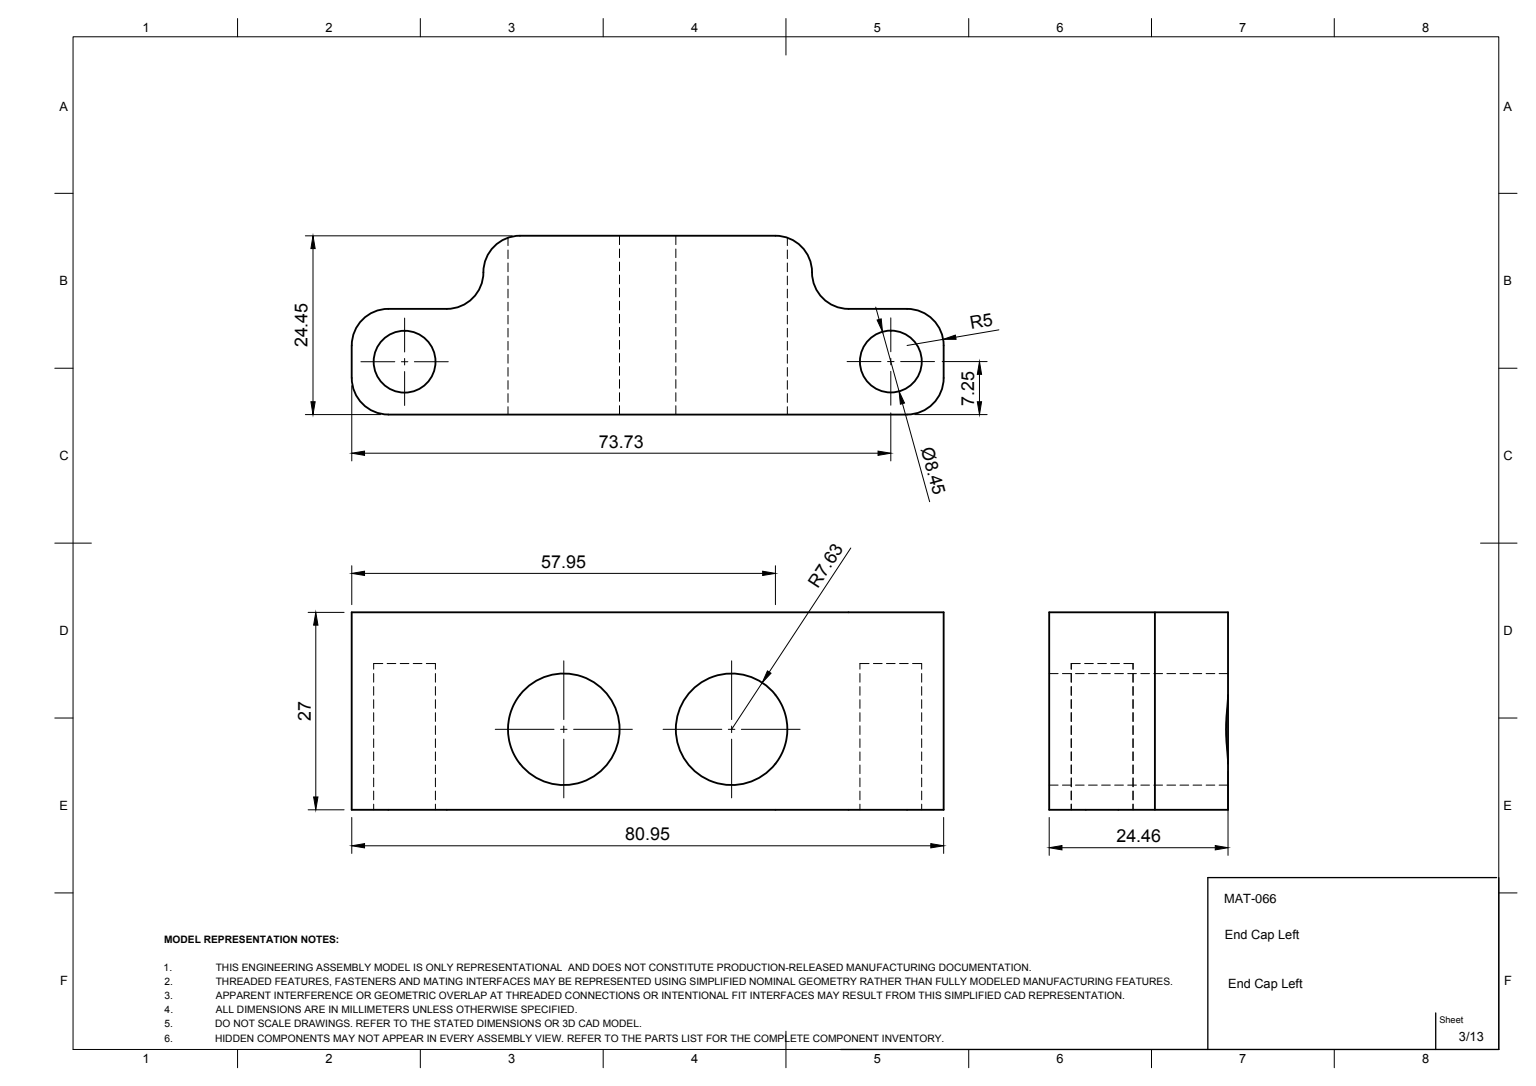
ISO-10303-21;
HEADER;
/* Generated by software containing ST-Developer
 * from STEP Tools, Inc. (www.steptools.com) 
 */

FILE_DESCRIPTION(
/* description */ ('CAx-IF Rec.Pracs.---Representation and Presentation of Product Manufa
cturing Information (PMI)---4.0---2014-10-13'),
/* implementation_level */ '2;1');

FILE_NAME(
/* name */ 'End Cap Left.step',
/* time_stamp */ '2026-10-24T15:58:00-07:00',
/* author */ (''),
/* organization */ (''),
/* preprocessor_version */ 'ST-DEVELOPER v20.2',
/* originating_system */ 'Autodesk Translation Framework v15.17.0.0',
/* authorisation */ '');

FILE_SCHEMA (('AP242_MANAGED_MODEL_BASED_3D_ENGINEERING_MIM_LF { 1 0 10303 442 2 1 4 }'));
ENDSEC;

DATA;
#10=MECHANICAL_DESIGN_GEOMETRIC_PRESENTATION_REPRESENTATION('',(#129),#8944);
#111=SHAPE_REPRESENTATION_RELATIONSHIP('SRR','None',#8993,#120);
#120=ADVANCED_BREP_SHAPE_REPRESENTATION('',(#138),#8934);
#129=STYLED_ITEM('',(#9052),#138);
#138=MANIFOLD_SOLID_BREP('Body1',#5150);
#147=B_SPLINE_CURVE_WITH_KNOTS('',3,(#7501,#7502,#7503,#7504,#7505,#7506),
 .UNSPECIFIED.,.F.,.F.,(4,2,4),(3.46797062946804,3.66737221611079,3.95578831781598),
 .UNSPECIFIED.);
#148=B_SPLINE_CURVE_WITH_KNOTS('',3,(#7507,#7508,#7509,#7510,#7511,#7512),
 .UNSPECIFIED.,.F.,.F.,(4,2,4),(3.95578831781598,4.24420441952117,4.44360600616391),
 .UNSPECIFIED.);
#149=B_SPLINE_CURVE_WITH_KNOTS('',3,(#7515,#7516,#7517,#7518,#7519,#7520,
#7521,#7522,#7523,#7524),.UNSPECIFIED.,.F.,.F.,(4,2,2,2,4),(-4.44360600616391,
-4.24420441952117,-3.95578831781597,-3.66737221611078,-3.46797062946804),
 .UNSPECIFIED.);
#153=CYLINDRICAL_SURFACE('',#5276,0.004225);
#154=CYLINDRICAL_SURFACE('',#5280,0.004225);
#155=CYLINDRICAL_SURFACE('',#5294,0.005);
#156=CYLINDRICAL_SURFACE('',#5295,0.005);
#157=CYLINDRICAL_SURFACE('',#5296,0.005);
#158=CYLINDRICAL_SURFACE('',#5297,0.005);
#159=CYLINDRICAL_SURFACE('',#5302,0.007625);
#160=CYLINDRICAL_SURFACE('',#5303,0.007625);
#161=CYLINDRICAL_SURFACE('',#5304,0.005);
#162=CYLINDRICAL_SURFACE('',#5305,0.005);
#163=CYLINDRICAL_SURFACE('',#5306,0.005);
#164=CYLINDRICAL_SURFACE('',#5307,0.005);
#238=FACE_BOUND('',#581,.T.);
#239=FACE_BOUND('',#582,.T.);
#240=FACE_BOUND('',#588,.T.);
#241=FACE_BOUND('',#589,.T.);
#308=FACE_OUTER_BOUND('',#577,.T.);
#309=FACE_OUTER_BOUND('',#578,.T.);
#310=FACE_OUTER_BOUND('',#579,.T.);
#311=FACE_OUTER_BOUND('',#580,.T.);
#312=FACE_OUTER_BOUND('',#583,.T.);
#313=FACE_OUTER_BOUND('',#584,.T.);
#314=FACE_OUTER_BOUND('',#585,.T.);
#315=FACE_OUTER_BOUND('',#586,.T.);
#316=FACE_OUTER_BOUND('',#587,.T.);
#317=FACE_OUTER_BOUND('',#590,.T.);
#318=FACE_OUTER_BOUND('',#591,.T.);
#319=FACE_OUTER_BOUND('',#592,.T.);
#320=FACE_OUTER_BOUND('',#593,.T.);
#321=FACE_OUTER_BOUND('',#594,.T.);
#322=FACE_OUTER_BOUND('',#595,.T.);
#323=FACE_OUTER_BOUND('',#596,.T.);
#324=FACE_OUTER_BOUND('',#597,.T.);
#325=FACE_OUTER_BOUND('',#598,.T.);
#326=FACE_OUTER_BOUND('',#599,.T.);
#327=FACE_OUTER_BOUND('',#600,.T.);
#328=FACE_OUTER_BOUND('',#601,.T.);
#329=FACE_OUTER_BOUND('',#602,.T.);
#577=EDGE_LOOP('',(#3275,#3276,#3277,#3278,#3279,#3280,#3281,#3282,#3283,
#3284,#3285,#3286,#3287,#3288));
#578=EDGE_LOOP('',(#3289,#3290,#3291,#3292));
#579=EDGE_LOOP('',(#3293,#3294,#3295,#3296));
#580=EDGE_LOOP('',(#3297,#3298,#3299,#3300));
#581=EDGE_LOOP('',(#3301));
#582=EDGE_LOOP('',(#3302));
#583=EDGE_LOOP('',(#3303,#3304,#3305,#3306));
#584=EDGE_LOOP('',(#3307,#3308,#3309,#3310));
#585=EDGE_LOOP('',(#3311,#3312,#3313,#3314));
#586=EDGE_LOOP('',(#3315,#3316,#3317,#3318));
#587=EDGE_LOOP('',(#3319,#3320,#3321,#3322,#3323,#3324,#3325,#3326,#3327,
#3328,#3329,#3330,#3331,#3332));
#588=EDGE_LOOP('',(#3333));
#589=EDGE_LOOP('',(#3334));
#590=EDGE_LOOP('',(#3335));
#591=EDGE_LOOP('',(#3336));
#592=EDGE_LOOP('',(#3337,#3338,#3339,#3340));
#593=EDGE_LOOP('',(#3341,#3342,#3343,#3344));
#594=EDGE_LOOP('',(#3345,#3346,#3347,#3348));
#595=EDGE_LOOP('',(#3349,#3350,#3351,#3352));
#596=EDGE_LOOP('',(#3353,#3354,#3355,#3356,#3357,#3358,#3359,#3360,#3361));
#597=EDGE_LOOP('',(#3362,#3363,#3364,#3365,#3366,#3367));
#598=EDGE_LOOP('',(#3368,#3369,#3370,#3371,#3372,#3373));
#599=EDGE_LOOP('',(#3374,#3375,#3376,#3377,#3378,#3379));
#600=EDGE_LOOP('',(#3380,#3381,#3382,#3383));
#601=EDGE_LOOP('',(#3384,#3385,#3386,#3387,#3388,#3389,#3390));
#602=EDGE_LOOP('',(#3391,#3392,#3393,#3394));
#916=CIRCLE('',#5262,0.00499999999999998);
#917=CIRCLE('',#5263,0.005);
#918=CIRCLE('',#5264,0.005);
#919=CIRCLE('',#5265,0.005);
#920=CIRCLE('',#5266,0.00500000000000002);
#921=CIRCLE('',#5267,0.00499999999999998);
#922=CIRCLE('',#5268,0.00500000000000002);
#923=CIRCLE('',#5269,0.00500000000000002);
#924=CIRCLE('',#5273,0.007625);
#925=CIRCLE('',#5274,0.007625);
#926=CIRCLE('',#5277,0.004225);
#927=CIRCLE('',#5278,0.004225);
#928=CIRCLE('',#5281,0.004225);
#929=CIRCLE('',#5282,0.004225);
#930=CIRCLE('',#5284,0.005);
#931=CIRCLE('',#5285,0.005);
#932=CIRCLE('',#5286,0.005);
#933=CIRCLE('',#5287,0.005);
#934=CIRCLE('',#5288,0.005);
#935=CIRCLE('',#5289,0.005);
#936=CIRCLE('',#5290,0.005);
#937=CIRCLE('',#5291,0.005);
#938=CIRCLE('',#5299,0.007625);
#939=CIRCLE('',#5300,0.007625);
#940=CIRCLE('',#5301,0.007625);
#1172=LINE('',#7393,#1627);
#1173=LINE('',#7397,#1628);
#1174=LINE('',#7401,#1629);
#1175=LINE('',#7405,#1630);
#1176=LINE('',#7409,#1631);
#1177=LINE('',#7415,#1632);
#1178=LINE('',#7422,#1633);
#1179=LINE('',#7423,#1634);
#1180=LINE('',#7424,#1635);
#1181=LINE('',#7427,#1636);
#1182=LINE('',#7429,#1637);
#1183=LINE('',#7430,#1638);
#1184=LINE('',#7433,#1639);
#1185=LINE('',#7435,#1640);
#1186=LINE('',#7436,#1641);
#1187=LINE('',#7443,#1642);
#1188=LINE('',#7445,#1643);
#1189=LINE('',#7446,#1644);
#1190=LINE('',#7451,#1645);
#1191=LINE('',#7455,#1646);
#1192=LINE('',#7457,#1647);
#1193=LINE('',#7458,#1648);
#1194=LINE('',#7463,#1649);
#1195=LINE('',#7468,#1650);
#1196=LINE('',#7487,#1651);
#1197=LINE('',#7492,#1652);
#1198=LINE('',#7494,#1653);
#1199=LINE('',#7497,#1654);
#1200=LINE('',#7500,#1655);
#1201=LINE('',#7514,#1656);
#1202=LINE('',#7526,#1657);
#1203=LINE('',#7529,#1658);
#1627=VECTOR('',#5823,0.01);
#1628=VECTOR('',#5826,0.01);
#1629=VECTOR('',#5829,0.01);
#1630=VECTOR('',#5832,0.01);
#1631=VECTOR('',#5835,0.01);
#1632=VECTOR('',#5840,0.01);
#1633=VECTOR('',#5847,1.);
#1634=VECTOR('',#5848,1.);
#1635=VECTOR('',#5849,1.);
#1636=VECTOR('',#5852,1.);
#1637=VECTOR('',#5853,1.);
#1638=VECTOR('',#5854,0.01);
#1639=VECTOR('',#5857,1.);
#1640=VECTOR('',#5858,1.);
#1641=VECTOR('',#5859,0.01);
#1642=VECTOR('',#5866,1.);
#1643=VECTOR('',#5867,1.);
#1644=VECTOR('',#5868,0.01);
#1645=VECTOR('',#5873,0.004225);
#1646=VECTOR('',#5878,1.);
#1647=VECTOR('',#5879,1.);
#1648=VECTOR('',#5880,0.01);
#1649=VECTOR('',#5885,0.004225);
#1650=VECTOR('',#5890,1.);
#1651=VECTOR('',#5921,0.01);
#1652=VECTOR('',#5926,1.);
#1653=VECTOR('',#5927,1.);
#1654=VECTOR('',#5930,0.01);
#1655=VECTOR('',#5933,0.007625);
#1656=VECTOR('',#5936,0.007625);
#1657=VECTOR('',#5939,0.01);
#1658=VECTOR('',#5944,0.01);
#2082=VERTEX_POINT('',#7391);
#2083=VERTEX_POINT('',#7392);
#2084=VERTEX_POINT('',#7394);
#2085=VERTEX_POINT('',#7396);
#2086=VERTEX_POINT('',#7398);
#2087=VERTEX_POINT('',#7400);
#2088=VERTEX_POINT('',#7402);
#2089=VERTEX_POINT('',#7404);
#2090=VERTEX_POINT('',#7406);
#2091=VERTEX_POINT('',#7408);
#2092=VERTEX_POINT('',#7410);
#2093=VERTEX_POINT('',#7412);
#2094=VERTEX_POINT('',#7414);
#2095=VERTEX_POINT('',#7416);
#2096=VERTEX_POINT('',#7420);
#2097=VERTEX_POINT('',#7421);
#2098=VERTEX_POINT('',#7426);
#2099=VERTEX_POINT('',#7428);
#2100=VERTEX_POINT('',#7432);
#2101=VERTEX_POINT('',#7434);
#2102=VERTEX_POINT('',#7437);
#2103=VERTEX_POINT('',#7439);
#2104=VERTEX_POINT('',#7442);
#2105=VERTEX_POINT('',#7444);
#2106=VERTEX_POINT('',#7448);
#2107=VERTEX_POINT('',#7450);
#2108=VERTEX_POINT('',#7454);
#2109=VERTEX_POINT('',#7456);
#2110=VERTEX_POINT('',#7460);
#2111=VERTEX_POINT('',#7462);
#2112=VERTEX_POINT('',#7466);
#2113=VERTEX_POINT('',#7467);
#2114=VERTEX_POINT('',#7469);
#2115=VERTEX_POINT('',#7476);
#2116=VERTEX_POINT('',#7486);
#2117=VERTEX_POINT('',#7488);
#2118=VERTEX_POINT('',#7490);
#2119=VERTEX_POINT('',#7493);
#2120=VERTEX_POINT('',#7495);
#2121=VERTEX_POINT('',#7499);
#2558=EDGE_CURVE('',#2082,#2083,#1172,.T.);
#2559=EDGE_CURVE('',#2083,#2084,#916,.T.);
#2560=EDGE_CURVE('',#2084,#2085,#1173,.T.);
#2561=EDGE_CURVE('',#2085,#2086,#917,.T.);
#2562=EDGE_CURVE('',#2086,#2087,#1174,.T.);
#2563=EDGE_CURVE('',#2087,#2088,#918,.T.);
#2564=EDGE_CURVE('',#2088,#2089,#1175,.T.);
#2565=EDGE_CURVE('',#2089,#2090,#919,.T.);
#2566=EDGE_CURVE('',#2090,#2091,#1176,.T.);
#2567=EDGE_CURVE('',#2091,#2092,#920,.T.);
#2568=EDGE_CURVE('',#2092,#2093,#921,.T.);
#2569=EDGE_CURVE('',#2093,#2094,#1177,.T.);
#2570=EDGE_CURVE('',#2094,#2095,#922,.T.);
#2571=EDGE_CURVE('',#2095,#2082,#923,.T.);
#2572=EDGE_CURVE('',#2096,#2097,#1178,.T.);
#2573=EDGE_CURVE('',#2096,#2091,#1179,.F.);
#2574=EDGE_CURVE('',#2090,#2097,#1180,.T.);
#2575=EDGE_CURVE('',#2084,#2098,#1181,.T.);
#2576=EDGE_CURVE('',#2099,#2098,#1182,.T.);
#2577=EDGE_CURVE('',#2099,#2085,#1183,.T.);
#2578=EDGE_CURVE('',#2086,#2100,#1184,.T.);
#2579=EDGE_CURVE('',#2100,#2101,#1185,.T.);
#2580=EDGE_CURVE('',#2101,#2087,#1186,.T.);
#2581=EDGE_CURVE('',#2102,#2102,#924,.T.);
#2582=EDGE_CURVE('',#2103,#2103,#925,.T.);
#2583=EDGE_CURVE('',#2088,#2104,#1187,.T.);
#2584=EDGE_CURVE('',#2104,#2105,#1188,.T.);
#2585=EDGE_CURVE('',#2105,#2089,#1189,.T.);
#2586=EDGE_CURVE('',#2106,#2106,#926,.T.);
#2587=EDGE_CURVE('',#2106,#2107,#1190,.T.);
#2588=EDGE_CURVE('',#2107,#2107,#927,.T.);
#2589=EDGE_CURVE('',#2082,#2108,#1191,.T.);
#2590=EDGE_CURVE('',#2109,#2108,#1192,.T.);
#2591=EDGE_CURVE('',#2109,#2083,#1193,.T.);
#2592=EDGE_CURVE('',#2110,#2110,#928,.T.);
#2593=EDGE_CURVE('',#2110,#2111,#1194,.T.);
#2594=EDGE_CURVE('',#2111,#2111,#929,.T.);
#2595=EDGE_CURVE('',#2112,#2113,#1195,.T.);
#2596=EDGE_CURVE('',#2113,#2114,#930,.F.);
#2597=EDGE_CURVE('',#2114,#2096,#931,.T.);
#2598=EDGE_CURVE('',#2097,#2105,#932,.F.);
#2599=EDGE_CURVE('',#2104,#2101,#933,.F.);
#2600=EDGE_CURVE('',#2100,#2099,#934,.F.);
#2601=EDGE_CURVE('',#2098,#2109,#935,.F.);
#2602=EDGE_CURVE('',#2108,#2115,#936,.T.);
#2603=EDGE_CURVE('',#2115,#2112,#937,.F.);
#2604=EDGE_CURVE('',#2116,#2093,#1196,.T.);
#2605=EDGE_CURVE('',#2117,#2116,#938,.T.);
#2606=EDGE_CURVE('',#2118,#2117,#939,.T.);
#2607=EDGE_CURVE('',#2118,#2113,#1197,.T.);
#2608=EDGE_CURVE('',#2112,#2119,#1198,.F.);
#2609=EDGE_CURVE('',#2120,#2119,#940,.T.);
#2610=EDGE_CURVE('',#2120,#2094,#1199,.T.);
#2611=EDGE_CURVE('',#2103,#2121,#1200,.T.);
#2612=EDGE_CURVE('',#2121,#2120,#147,.F.);
#2613=EDGE_CURVE('',#2119,#2121,#148,.F.);
#2614=EDGE_CURVE('',#2102,#2117,#1201,.T.);
#2615=EDGE_CURVE('',#2116,#2118,#149,.T.);
#2616=EDGE_CURVE('',#2114,#2092,#1202,.T.);
#2617=EDGE_CURVE('',#2115,#2095,#1203,.T.);
#3275=ORIENTED_EDGE('',*,*,#2558,.T.);
#3276=ORIENTED_EDGE('',*,*,#2559,.T.);
#3277=ORIENTED_EDGE('',*,*,#2560,.T.);
#3278=ORIENTED_EDGE('',*,*,#2561,.T.);
#3279=ORIENTED_EDGE('',*,*,#2562,.T.);
#3280=ORIENTED_EDGE('',*,*,#2563,.T.);
#3281=ORIENTED_EDGE('',*,*,#2564,.T.);
#3282=ORIENTED_EDGE('',*,*,#2565,.T.);
#3283=ORIENTED_EDGE('',*,*,#2566,.T.);
#3284=ORIENTED_EDGE('',*,*,#2567,.T.);
#3285=ORIENTED_EDGE('',*,*,#2568,.T.);
#3286=ORIENTED_EDGE('',*,*,#2569,.T.);
#3287=ORIENTED_EDGE('',*,*,#2570,.T.);
#3288=ORIENTED_EDGE('',*,*,#2571,.T.);
#3289=ORIENTED_EDGE('',*,*,#2572,.F.);
#3290=ORIENTED_EDGE('',*,*,#2573,.T.);
#3291=ORIENTED_EDGE('',*,*,#2566,.F.);
#3292=ORIENTED_EDGE('',*,*,#2574,.T.);
#3293=ORIENTED_EDGE('',*,*,#2575,.T.);
#3294=ORIENTED_EDGE('',*,*,#2576,.F.);
#3295=ORIENTED_EDGE('',*,*,#2577,.T.);
#3296=ORIENTED_EDGE('',*,*,#2560,.F.);
#3297=ORIENTED_EDGE('',*,*,#2578,.T.);
#3298=ORIENTED_EDGE('',*,*,#2579,.T.);
#3299=ORIENTED_EDGE('',*,*,#2580,.T.);
#3300=ORIENTED_EDGE('',*,*,#2562,.F.);
#3301=ORIENTED_EDGE('',*,*,#2581,.T.);
#3302=ORIENTED_EDGE('',*,*,#2582,.T.);
#3303=ORIENTED_EDGE('',*,*,#2583,.T.);
#3304=ORIENTED_EDGE('',*,*,#2584,.T.);
#3305=ORIENTED_EDGE('',*,*,#2585,.T.);
#3306=ORIENTED_EDGE('',*,*,#2564,.F.);
#3307=ORIENTED_EDGE('',*,*,#2586,.T.);
#3308=ORIENTED_EDGE('',*,*,#2587,.T.);
#3309=ORIENTED_EDGE('',*,*,#2588,.F.);
#3310=ORIENTED_EDGE('',*,*,#2587,.F.);
#3311=ORIENTED_EDGE('',*,*,#2589,.T.);
#3312=ORIENTED_EDGE('',*,*,#2590,.F.);
#3313=ORIENTED_EDGE('',*,*,#2591,.T.);
#3314=ORIENTED_EDGE('',*,*,#2558,.F.);
#3315=ORIENTED_EDGE('',*,*,#2592,.T.);
#3316=ORIENTED_EDGE('',*,*,#2593,.T.);
#3317=ORIENTED_EDGE('',*,*,#2594,.F.);
#3318=ORIENTED_EDGE('',*,*,#2593,.F.);
#3319=ORIENTED_EDGE('',*,*,#2595,.T.);
#3320=ORIENTED_EDGE('',*,*,#2596,.T.);
#3321=ORIENTED_EDGE('',*,*,#2597,.T.);
#3322=ORIENTED_EDGE('',*,*,#2572,.T.);
#3323=ORIENTED_EDGE('',*,*,#2598,.T.);
#3324=ORIENTED_EDGE('',*,*,#2584,.F.);
#3325=ORIENTED_EDGE('',*,*,#2599,.T.);
#3326=ORIENTED_EDGE('',*,*,#2579,.F.);
#3327=ORIENTED_EDGE('',*,*,#2600,.T.);
#3328=ORIENTED_EDGE('',*,*,#2576,.T.);
#3329=ORIENTED_EDGE('',*,*,#2601,.T.);
#3330=ORIENTED_EDGE('',*,*,#2590,.T.);
#3331=ORIENTED_EDGE('',*,*,#2602,.T.);
#3332=ORIENTED_EDGE('',*,*,#2603,.T.);
#3333=ORIENTED_EDGE('',*,*,#2588,.T.);
#3334=ORIENTED_EDGE('',*,*,#2594,.T.);
#3335=ORIENTED_EDGE('',*,*,#2592,.F.);
#3336=ORIENTED_EDGE('',*,*,#2586,.F.);
#3337=ORIENTED_EDGE('',*,*,#2591,.F.);
#3338=ORIENTED_EDGE('',*,*,#2601,.F.);
#3339=ORIENTED_EDGE('',*,*,#2575,.F.);
#3340=ORIENTED_EDGE('',*,*,#2559,.F.);
#3341=ORIENTED_EDGE('',*,*,#2577,.F.);
#3342=ORIENTED_EDGE('',*,*,#2600,.F.);
#3343=ORIENTED_EDGE('',*,*,#2578,.F.);
#3344=ORIENTED_EDGE('',*,*,#2561,.F.);
#3345=ORIENTED_EDGE('',*,*,#2580,.F.);
#3346=ORIENTED_EDGE('',*,*,#2599,.F.);
#3347=ORIENTED_EDGE('',*,*,#2583,.F.);
#3348=ORIENTED_EDGE('',*,*,#2563,.F.);
#3349=ORIENTED_EDGE('',*,*,#2585,.F.);
#3350=ORIENTED_EDGE('',*,*,#2598,.F.);
#3351=ORIENTED_EDGE('',*,*,#2574,.F.);
#3352=ORIENTED_EDGE('',*,*,#2565,.F.);
#3353=ORIENTED_EDGE('',*,*,#2604,.F.);
#3354=ORIENTED_EDGE('',*,*,#2605,.F.);
#3355=ORIENTED_EDGE('',*,*,#2606,.F.);
#3356=ORIENTED_EDGE('',*,*,#2607,.T.);
#3357=ORIENTED_EDGE('',*,*,#2595,.F.);
#3358=ORIENTED_EDGE('',*,*,#2608,.T.);
#3359=ORIENTED_EDGE('',*,*,#2609,.F.);
#3360=ORIENTED_EDGE('',*,*,#2610,.T.);
#3361=ORIENTED_EDGE('',*,*,#2569,.F.);
#3362=ORIENTED_EDGE('',*,*,#2582,.F.);
#3363=ORIENTED_EDGE('',*,*,#2611,.T.);
#3364=ORIENTED_EDGE('',*,*,#2612,.T.);
#3365=ORIENTED_EDGE('',*,*,#2609,.T.);
#3366=ORIENTED_EDGE('',*,*,#2613,.T.);
#3367=ORIENTED_EDGE('',*,*,#2611,.F.);
#3368=ORIENTED_EDGE('',*,*,#2581,.F.);
#3369=ORIENTED_EDGE('',*,*,#2614,.T.);
#3370=ORIENTED_EDGE('',*,*,#2605,.T.);
#3371=ORIENTED_EDGE('',*,*,#2615,.T.);
#3372=ORIENTED_EDGE('',*,*,#2606,.T.);
#3373=ORIENTED_EDGE('',*,*,#2614,.F.);
#3374=ORIENTED_EDGE('',*,*,#2604,.T.);
#3375=ORIENTED_EDGE('',*,*,#2568,.F.);
#3376=ORIENTED_EDGE('',*,*,#2616,.F.);
#3377=ORIENTED_EDGE('',*,*,#2596,.F.);
#3378=ORIENTED_EDGE('',*,*,#2607,.F.);
#3379=ORIENTED_EDGE('',*,*,#2615,.F.);
#3380=ORIENTED_EDGE('',*,*,#2573,.F.);
#3381=ORIENTED_EDGE('',*,*,#2597,.F.);
#3382=ORIENTED_EDGE('',*,*,#2616,.T.);
#3383=ORIENTED_EDGE('',*,*,#2567,.F.);
#3384=ORIENTED_EDGE('',*,*,#2617,.T.);
#3385=ORIENTED_EDGE('',*,*,#2570,.F.);
#3386=ORIENTED_EDGE('',*,*,#2610,.F.);
#3387=ORIENTED_EDGE('',*,*,#2612,.F.);
#3388=ORIENTED_EDGE('',*,*,#2613,.F.);
#3389=ORIENTED_EDGE('',*,*,#2608,.F.);
#3390=ORIENTED_EDGE('',*,*,#2603,.F.);
#3391=ORIENTED_EDGE('',*,*,#2617,.F.);
#3392=ORIENTED_EDGE('',*,*,#2602,.F.);
#3393=ORIENTED_EDGE('',*,*,#2589,.F.);
#3394=ORIENTED_EDGE('',*,*,#2571,.F.);
#4709=PLANE('',#5261);
#4710=PLANE('',#5270);
#4711=PLANE('',#5271);
#4712=PLANE('',#5272);
#4713=PLANE('',#5275);
#4714=PLANE('',#5279);
#4715=PLANE('',#5283);
#4716=PLANE('',#5292);
#4717=PLANE('',#5293);
#4718=PLANE('',#5298);
#4881=ADVANCED_FACE('',(#308),#4709,.T.);
#4882=ADVANCED_FACE('',(#309),#4710,.T.);
#4883=ADVANCED_FACE('',(#310),#4711,.T.);
#4884=ADVANCED_FACE('',(#311,#238,#239),#4712,.F.);
#4885=ADVANCED_FACE('',(#312),#4713,.F.);
#4886=ADVANCED_FACE('',(#313),#153,.F.);
#4887=ADVANCED_FACE('',(#314),#4714,.T.);
#4888=ADVANCED_FACE('',(#315),#154,.F.);
#4889=ADVANCED_FACE('',(#316,#240,#241),#4715,.F.);
#4890=ADVANCED_FACE('',(#317),#4716,.F.);
#4891=ADVANCED_FACE('',(#318),#4717,.F.);
#4892=ADVANCED_FACE('',(#319),#155,.T.);
#4893=ADVANCED_FACE('',(#320),#156,.T.);
#4894=ADVANCED_FACE('',(#321),#157,.T.);
#4895=ADVANCED_FACE('',(#322),#158,.T.);
#4896=ADVANCED_FACE('',(#323),#4718,.T.);
#4897=ADVANCED_FACE('',(#324),#159,.F.);
#4898=ADVANCED_FACE('',(#325),#160,.F.);
#4899=ADVANCED_FACE('',(#326),#161,.T.);
#4900=ADVANCED_FACE('',(#327),#162,.F.);
#4901=ADVANCED_FACE('',(#328),#163,.T.);
#4902=ADVANCED_FACE('',(#329),#164,.F.);
#5150=CLOSED_SHELL('',(#4881,#4882,#4883,#4884,#4885,#4886,#4887,#4888,
#4889,#4890,#4891,#4892,#4893,#4894,#4895,#4896,#4897,#4898,#4899,#4900,
#4901,#4902));
#5260=AXIS2_PLACEMENT_3D('',#7389,#5819,#5820);
#5261=AXIS2_PLACEMENT_3D('',#7390,#5821,#5822);
#5262=AXIS2_PLACEMENT_3D('',#7395,#5824,#5825);
#5263=AXIS2_PLACEMENT_3D('',#7399,#5827,#5828);
#5264=AXIS2_PLACEMENT_3D('',#7403,#5830,#5831);
#5265=AXIS2_PLACEMENT_3D('',#7407,#5833,#5834);
#5266=AXIS2_PLACEMENT_3D('',#7411,#5836,#5837);
#5267=AXIS2_PLACEMENT_3D('',#7413,#5838,#5839);
#5268=AXIS2_PLACEMENT_3D('',#7417,#5841,#5842);
#5269=AXIS2_PLACEMENT_3D('',#7418,#5843,#5844);
#5270=AXIS2_PLACEMENT_3D('',#7419,#5845,#5846);
#5271=AXIS2_PLACEMENT_3D('',#7425,#5850,#5851);
#5272=AXIS2_PLACEMENT_3D('',#7431,#5855,#5856);
#5273=AXIS2_PLACEMENT_3D('',#7438,#5860,#5861);
#5274=AXIS2_PLACEMENT_3D('',#7440,#5862,#5863);
#5275=AXIS2_PLACEMENT_3D('',#7441,#5864,#5865);
#5276=AXIS2_PLACEMENT_3D('',#7447,#5869,#5870);
#5277=AXIS2_PLACEMENT_3D('',#7449,#5871,#5872);
#5278=AXIS2_PLACEMENT_3D('',#7452,#5874,#5875);
#5279=AXIS2_PLACEMENT_3D('',#7453,#5876,#5877);
#5280=AXIS2_PLACEMENT_3D('',#7459,#5881,#5882);
#5281=AXIS2_PLACEMENT_3D('',#7461,#5883,#5884);
#5282=AXIS2_PLACEMENT_3D('',#7464,#5886,#5887);
#5283=AXIS2_PLACEMENT_3D('',#7465,#5888,#5889);
#5284=AXIS2_PLACEMENT_3D('',#7470,#5891,#5892);
#5285=AXIS2_PLACEMENT_3D('',#7471,#5893,#5894);
#5286=AXIS2_PLACEMENT_3D('',#7472,#5895,#5896);
#5287=AXIS2_PLACEMENT_3D('',#7473,#5897,#5898);
#5288=AXIS2_PLACEMENT_3D('',#7474,#5899,#5900);
#5289=AXIS2_PLACEMENT_3D('',#7475,#5901,#5902);
#5290=AXIS2_PLACEMENT_3D('',#7477,#5903,#5904);
#5291=AXIS2_PLACEMENT_3D('',#7478,#5905,#5906);
#5292=AXIS2_PLACEMENT_3D('',#7479,#5907,#5908);
#5293=AXIS2_PLACEMENT_3D('',#7480,#5909,#5910);
#5294=AXIS2_PLACEMENT_3D('',#7481,#5911,#5912);
#5295=AXIS2_PLACEMENT_3D('',#7482,#5913,#5914);
#5296=AXIS2_PLACEMENT_3D('',#7483,#5915,#5916);
#5297=AXIS2_PLACEMENT_3D('',#7484,#5917,#5918);
#5298=AXIS2_PLACEMENT_3D('',#7485,#5919,#5920);
#5299=AXIS2_PLACEMENT_3D('',#7489,#5922,#5923);
#5300=AXIS2_PLACEMENT_3D('',#7491,#5924,#5925);
#5301=AXIS2_PLACEMENT_3D('',#7496,#5928,#5929);
#5302=AXIS2_PLACEMENT_3D('',#7498,#5931,#5932);
#5303=AXIS2_PLACEMENT_3D('',#7513,#5934,#5935);
#5304=AXIS2_PLACEMENT_3D('',#7525,#5937,#5938);
#5305=AXIS2_PLACEMENT_3D('',#7527,#5940,#5941);
#5306=AXIS2_PLACEMENT_3D('',#7528,#5942,#5943);
#5307=AXIS2_PLACEMENT_3D('',#7530,#5945,#5946);
#5819=DIRECTION('axis',(0.,0.,1.));
#5820=DIRECTION('refdir',(1.,0.,0.));
#5821=DIRECTION('center_axis',(-1.,1.34377255958835E-12,4.29697613365962E-25));
#5822=DIRECTION('ref_axis',(-1.34377255958835E-12,-1.,8.56382801334526E-17));
#5823=DIRECTION('',(-4.23473790744943E-21,-2.13480776911686E-15,1.));
#5824=DIRECTION('center_axis',(-1.,1.34421664202194E-12,4.29697613365962E-25));
#5825=DIRECTION('ref_axis',(-1.34421664202194E-12,-1.,8.56382801334526E-17));
#5826=DIRECTION('',(1.34377255958835E-12,1.,-8.56382801334526E-17));
#5827=DIRECTION('center_axis',(-1.,1.34377255958835E-12,4.44095986543338E-16));
#5828=DIRECTION('ref_axis',(4.44095986553001E-16,7.19106563773386E-15,1.));
#5829=DIRECTION('',(-4.77967767461644E-22,-8.56382801334526E-17,-1.));
#5830=DIRECTION('center_axis',(-1.,1.34332846360224E-12,4.2969924039158E-25));
#5831=DIRECTION('ref_axis',(1.34332846360224E-12,1.,-3.63835195893395E-15));
#5832=DIRECTION('',(-1.34377255958835E-12,-1.,8.56382801334526E-17));
#5833=DIRECTION('center_axis',(-1.,1.34377255958835E-12,6.77669327569707E-21));
#5834=DIRECTION('ref_axis',(-6.77670293885375E-21,-7.19106563773446E-15,
-1.));
#5835=DIRECTION('',(4.29812688450512E-25,8.56382801334526E-17,1.));
#5836=DIRECTION('center_axis',(1.,-1.34377255958835E-12,-4.29697613365962E-25));
#5837=DIRECTION('ref_axis',(4.34586730890502E-25,3.63835195893394E-15,1.));
#5838=DIRECTION('center_axis',(-1.,1.34377255958835E-12,4.29697613365962E-25));
#5839=DIRECTION('ref_axis',(-4.29812691736856E-25,-8.56382801334526E-17,
-1.));
#5840=DIRECTION('',(9.69851673070364E-22,-4.22618326275775E-16,1.));
#5841=DIRECTION('center_axis',(-1.,1.34377255281209E-12,4.29697613365962E-25));
#5842=DIRECTION('ref_axis',(-1.34377255281209E-12,-1.,8.56382801334526E-17));
#5843=DIRECTION('center_axis',(1.,-1.34377255958835E-12,-4.29697613365962E-25));
#5844=DIRECTION('ref_axis',(1.34377255958835E-12,1.,-7.19106563773443E-15));
#5845=DIRECTION('center_axis',(0.,-1.,8.57182693503055E-17));
#5846=DIRECTION('ref_axis',(0.,-8.57182693503055E-17,-1.));
#5847=DIRECTION('',(0.,-8.57182693503055E-17,-1.));
#5848=DIRECTION('',(1.,0.,0.));
#5849=DIRECTION('',(1.,0.,0.));
#5850=DIRECTION('center_axis',(0.,0.,1.));
#5851=DIRECTION('ref_axis',(1.,0.,0.));
#5852=DIRECTION('',(1.,0.,0.));
#5853=DIRECTION('',(0.,-1.,0.));
#5854=DIRECTION('',(-1.,1.34381394900629E-12,0.));
#5855=DIRECTION('center_axis',(0.,-1.,6.42887020127291E-17));
#5856=DIRECTION('ref_axis',(0.,-6.42887020127291E-17,-1.));
#5857=DIRECTION('',(1.,0.,0.));
#5858=DIRECTION('',(0.,-6.42887020127291E-17,-1.));
#5859=DIRECTION('',(-1.,1.34381394900629E-12,0.));
#5860=DIRECTION('center_axis',(0.,-1.,6.42887020127291E-17));
#5861=DIRECTION('ref_axis',(0.,-6.42887020127291E-17,-1.));
#5862=DIRECTION('center_axis',(0.,-1.,6.42887020127291E-17));
#5863=DIRECTION('ref_axis',(0.,-6.42887020127291E-17,-1.));
#5864=DIRECTION('center_axis',(0.,0.,1.));
#5865=DIRECTION('ref_axis',(1.,0.,0.));
#5866=DIRECTION('',(1.,0.,0.));
#5867=DIRECTION('',(0.,-1.,0.));
#5868=DIRECTION('',(-1.,1.34381394900629E-12,0.));
#5869=DIRECTION('center_axis',(1.,0.,0.));
#5870=DIRECTION('ref_axis',(0.,0.,-1.));
#5871=DIRECTION('center_axis',(-1.,0.,0.));
#5872=DIRECTION('ref_axis',(0.,0.,1.));
#5873=DIRECTION('',(1.,0.,0.));
#5874=DIRECTION('center_axis',(-1.,0.,0.));
#5875=DIRECTION('ref_axis',(0.,0.,1.));
#5876=DIRECTION('center_axis',(0.,-1.,8.57182693503055E-17));
#5877=DIRECTION('ref_axis',(0.,-8.57182693503055E-17,-1.));
#5878=DIRECTION('',(1.,0.,0.));
#5879=DIRECTION('',(0.,-8.57182693503055E-17,-1.));
#5880=DIRECTION('',(-1.,1.34381394900629E-12,0.));
#5881=DIRECTION('center_axis',(1.,0.,0.));
#5882=DIRECTION('ref_axis',(0.,0.,-1.));
#5883=DIRECTION('center_axis',(-1.,0.,0.));
#5884=DIRECTION('ref_axis',(0.,0.,1.));
#5885=DIRECTION('',(1.,0.,0.));
#5886=DIRECTION('center_axis',(-1.,0.,0.));
#5887=DIRECTION('ref_axis',(0.,0.,1.));
#5888=DIRECTION('center_axis',(-1.,0.,0.));
#5889=DIRECTION('ref_axis',(0.,-1.,0.));
#5890=DIRECTION('',(0.,-8.57182693503055E-17,-1.));
#5891=DIRECTION('center_axis',(-1.,0.,0.));
#5892=DIRECTION('ref_axis',(0.,0.,1.));
#5893=DIRECTION('center_axis',(-1.,0.,0.));
#5894=DIRECTION('ref_axis',(0.,0.,1.));
#5895=DIRECTION('center_axis',(-1.,0.,0.));
#5896=DIRECTION('ref_axis',(0.,0.,1.));
#5897=DIRECTION('center_axis',(-1.,0.,0.));
#5898=DIRECTION('ref_axis',(0.,0.,1.));
#5899=DIRECTION('center_axis',(-1.,0.,0.));
#5900=DIRECTION('ref_axis',(0.,0.,1.));
#5901=DIRECTION('center_axis',(-1.,0.,0.));
#5902=DIRECTION('ref_axis',(0.,0.,1.));
#5903=DIRECTION('center_axis',(-1.,0.,0.));
#5904=DIRECTION('ref_axis',(0.,0.,1.));
#5905=DIRECTION('center_axis',(-1.,0.,0.));
#5906=DIRECTION('ref_axis',(0.,0.,1.));
#5907=DIRECTION('center_axis',(-1.,0.,0.));
#5908=DIRECTION('ref_axis',(0.,-1.,0.));
#5909=DIRECTION('center_axis',(-1.,0.,0.));
#5910=DIRECTION('ref_axis',(0.,-1.,0.));
#5911=DIRECTION('center_axis',(1.,0.,0.));
#5912=DIRECTION('ref_axis',(0.,0.,-1.));
#5913=DIRECTION('center_axis',(-1.,0.,0.));
#5914=DIRECTION('ref_axis',(0.,0.,1.));
#5915=DIRECTION('center_axis',(1.,0.,0.));
#5916=DIRECTION('ref_axis',(0.,0.,-1.));
#5917=DIRECTION('center_axis',(-1.,0.,0.));
#5918=DIRECTION('ref_axis',(0.,0.,1.));
#5919=DIRECTION('center_axis',(0.,-1.,8.57182693503055E-17));
#5920=DIRECTION('ref_axis',(1.,0.,0.));
#5921=DIRECTION('',(-1.,1.34381394900629E-12,0.));
#5922=DIRECTION('center_axis',(0.,-1.,8.57182693503055E-17));
#5923=DIRECTION('ref_axis',(0.,-8.57182693503055E-17,-1.));
#5924=DIRECTION('center_axis',(0.,-1.,8.57182693503055E-17));
#5925=DIRECTION('ref_axis',(0.,-8.57182693503055E-17,-1.));
#5926=DIRECTION('',(1.,0.,0.));
#5927=DIRECTION('',(1.,0.,0.));
#5928=DIRECTION('center_axis',(0.,-1.,8.57182693503055E-17));
#5929=DIRECTION('ref_axis',(0.,-8.57182693503055E-17,-1.));
#5930=DIRECTION('',(-1.,1.34381394900629E-12,0.));
#5931=DIRECTION('center_axis',(0.,-1.,8.57182693503055E-17));
#5932=DIRECTION('ref_axis',(0.,-8.57182693503055E-17,-1.));
#5933=DIRECTION('',(0.,-1.,8.57182693503055E-17));
#5934=DIRECTION('center_axis',(0.,-1.,8.57182693503055E-17));
#5935=DIRECTION('ref_axis',(0.,-8.57182693503055E-17,-1.));
#5936=DIRECTION('',(0.,-1.,8.57182693503055E-17));
#5937=DIRECTION('center_axis',(-1.,0.,0.));
#5938=DIRECTION('ref_axis',(0.,0.,1.));
#5939=DIRECTION('',(-1.,1.34381394900629E-12,0.));
#5940=DIRECTION('center_axis',(1.,0.,0.));
#5941=DIRECTION('ref_axis',(0.,0.,-1.));
#5942=DIRECTION('center_axis',(1.,0.,0.));
#5943=DIRECTION('ref_axis',(0.,0.,-1.));
#5944=DIRECTION('',(-1.,1.34381394900629E-12,0.));
#5945=DIRECTION('center_axis',(-1.,0.,0.));
#5946=DIRECTION('ref_axis',(0.,0.,1.));
#7389=CARTESIAN_POINT('',(0.,0.,0.));
#7390=CARTESIAN_POINT('Origin',(-0.0735499999997847,-0.0149749999999933,
0.02565));
#7391=CARTESIAN_POINT('',(-0.0735499999997877,-0.0171999999999932,0.053125));
#7392=CARTESIAN_POINT('',(-0.0735499999997876,-0.0171999999999933,0.061125));
#7393=CARTESIAN_POINT('',(-0.0735499999997877,-0.0171999999999932,0.053125));
#7394=CARTESIAN_POINT('',(-0.0735499999997809,-0.0121999999999932,0.066125));
#7395=CARTESIAN_POINT('Origin',(-0.0735499999997809,-0.0121999999999932,
0.061125));
#7396=CARTESIAN_POINT('',(-0.073549999999775,-0.00774999999999323,0.066125));
#7397=CARTESIAN_POINT('',(-0.0735499999997809,-0.0121999999999932,0.066125));
#7398=CARTESIAN_POINT('',(-0.0735499999997682,-0.00274999999999323,0.061125));
#7399=CARTESIAN_POINT('Origin',(-0.073549999999775,-0.00774999999999327,
0.061125));
#7400=CARTESIAN_POINT('',(-0.0735499999997682,-0.00274999999999327,-0.009825));
#7401=CARTESIAN_POINT('',(-0.0735499999997682,-0.00274999999999323,0.061125));
#7402=CARTESIAN_POINT('',(-0.0735499999997749,-0.0077499999999933,-0.014825));
#7403=CARTESIAN_POINT('Origin',(-0.0735499999997749,-0.0077499999999933,
-0.00982499999999996));
#7404=CARTESIAN_POINT('',(-0.0735499999997809,-0.0121999999999933,-0.014825));
#7405=CARTESIAN_POINT('',(-0.0735499999997749,-0.0077499999999933,-0.014825));
#7406=CARTESIAN_POINT('',(-0.0735499999997876,-0.0171999999999933,-0.00982499999999996));
#7407=CARTESIAN_POINT('Origin',(-0.0735499999997809,-0.0121999999999933,
-0.00982499999999996));
#7408=CARTESIAN_POINT('',(-0.0735499999997877,-0.0171999999999932,-0.00182499999999996));
#7409=CARTESIAN_POINT('',(-0.0735499999997876,-0.0171999999999933,-0.00982499999999996));
#7410=CARTESIAN_POINT('',(-0.0735499999997944,-0.0221999999999932,0.00317500000000004));
#7411=CARTESIAN_POINT('Origin',(-0.0735499999997944,-0.0221999999999932,
-0.00182499999999997));
#7412=CARTESIAN_POINT('',(-0.0735499999998011,-0.0271999999999932,0.00817500000000003));
#7413=CARTESIAN_POINT('Origin',(-0.0735499999997944,-0.0221999999999932,
0.00817500000000003));
#7414=CARTESIAN_POINT('',(-0.0735499999998011,-0.0271999999999932,0.043125));
#7415=CARTESIAN_POINT('',(-0.0735499999998011,-0.0271999999999932,0.00817500000000003));
#7416=CARTESIAN_POINT('',(-0.0735499999997944,-0.0221999999999932,0.0481250000000001));
#7417=CARTESIAN_POINT('Origin',(-0.0735499999997944,-0.0221999999999932,
0.043125));
#7418=CARTESIAN_POINT('Origin',(-0.0735499999997944,-0.0221999999999932,
0.0531250000000001));
#7419=CARTESIAN_POINT('Origin',(-0.06655,-0.0172,0.02565));
#7420=CARTESIAN_POINT('',(-0.04655,-0.0172,-0.001825));
#7421=CARTESIAN_POINT('',(-0.04655,-0.0172,-0.009825));
#7422=CARTESIAN_POINT('',(-0.04655,-0.0172,0.02565));
#7423=CARTESIAN_POINT('',(-0.06655,-0.0172,-0.001825));
#7424=CARTESIAN_POINT('',(-0.04655,-0.0172,-0.009825));
#7425=CARTESIAN_POINT('Origin',(-0.06655,-0.009975,0.066125));
#7426=CARTESIAN_POINT('',(-0.04655,-0.0122,0.066125));
#7427=CARTESIAN_POINT('',(-0.06655,-0.0122,0.066125));
#7428=CARTESIAN_POINT('',(-0.04655,-0.00775,0.066125));
#7429=CARTESIAN_POINT('',(-0.04655,-0.009975,0.066125));
#7430=CARTESIAN_POINT('',(-0.068549999999775,-0.00774999999999995,0.066125));
#7431=CARTESIAN_POINT('Origin',(-0.06655,-0.00275,0.02565));
#7432=CARTESIAN_POINT('',(-0.04655,-0.00275,0.061125));
#7433=CARTESIAN_POINT('',(-0.04655,-0.00275,0.061125));
#7434=CARTESIAN_POINT('',(-0.04655,-0.00275,-0.009825));
#7435=CARTESIAN_POINT('',(-0.04655,-0.00275,0.02565));
#7436=CARTESIAN_POINT('',(-0.0685499999997682,-0.00274999999999999,-0.009825));
#7437=CARTESIAN_POINT('',(-0.05755,-0.00275,0.0218));
#7438=CARTESIAN_POINT('Origin',(-0.05755,-0.00275,0.014175));
#7439=CARTESIAN_POINT('',(-0.05755,-0.00275,0.04475));
#7440=CARTESIAN_POINT('Origin',(-0.05755,-0.00275,0.037125));
#7441=CARTESIAN_POINT('Origin',(-0.06655,-0.009975,-0.014825));
#7442=CARTESIAN_POINT('',(-0.04655,-0.00775,-0.014825));
#7443=CARTESIAN_POINT('',(-0.06655,-0.00775,-0.014825));
#7444=CARTESIAN_POINT('',(-0.04655,-0.0122,-0.014825));
#7445=CARTESIAN_POINT('',(-0.04655,-0.009975,-0.014825));
#7446=CARTESIAN_POINT('',(-0.0685499999997809,-0.0122,-0.014825));
#7447=CARTESIAN_POINT('Origin',(-0.06655,-0.009975,-0.0076));
#7448=CARTESIAN_POINT('',(-0.06655,-0.009975,-0.003375));
#7449=CARTESIAN_POINT('Origin',(-0.06655,-0.009975,-0.0076));
#7450=CARTESIAN_POINT('',(-0.04655,-0.009975,-0.003375));
#7451=CARTESIAN_POINT('',(-0.06655,-0.009975,-0.003375));
#7452=CARTESIAN_POINT('Origin',(-0.04655,-0.009975,-0.0076));
#7453=CARTESIAN_POINT('Origin',(-0.06655,-0.0172,0.02565));
#7454=CARTESIAN_POINT('',(-0.04655,-0.0172,0.053125));
#7455=CARTESIAN_POINT('',(-0.04655,-0.0172,0.053125));
#7456=CARTESIAN_POINT('',(-0.04655,-0.0172,0.061125));
#7457=CARTESIAN_POINT('',(-0.04655,-0.0172,0.02565));
#7458=CARTESIAN_POINT('',(-0.0685499999997877,-0.0172,0.061125));
#7459=CARTESIAN_POINT('Origin',(-0.06655,-0.01,0.0589));
#7460=CARTESIAN_POINT('',(-0.06655,-0.01,0.063125));
#7461=CARTESIAN_POINT('Origin',(-0.06655,-0.01,0.0589));
#7462=CARTESIAN_POINT('',(-0.04655,-0.01,0.063125));
#7463=CARTESIAN_POINT('',(-0.06655,-0.01,0.063125));
#7464=CARTESIAN_POINT('Origin',(-0.04655,-0.01,0.0589));
#7465=CARTESIAN_POINT('Origin',(-0.04655,0.,0.02565));
#7466=CARTESIAN_POINT('',(-0.04655,-0.0272,0.043125));
#7467=CARTESIAN_POINT('',(-0.04655,-0.0272,0.008175));
#7468=CARTESIAN_POINT('',(-0.04655,-0.0272,0.02565));
#7469=CARTESIAN_POINT('',(-0.04655,-0.0222,0.003175));
#7470=CARTESIAN_POINT('Origin',(-0.04655,-0.0222,0.008175));
#7471=CARTESIAN_POINT('Origin',(-0.04655,-0.0222,-0.001825));
#7472=CARTESIAN_POINT('Origin',(-0.04655,-0.0122,-0.009825));
#7473=CARTESIAN_POINT('Origin',(-0.04655,-0.00775,-0.009825));
#7474=CARTESIAN_POINT('Origin',(-0.04655,-0.00775,0.061125));
#7475=CARTESIAN_POINT('Origin',(-0.04655,-0.0122,0.061125));
#7476=CARTESIAN_POINT('',(-0.04655,-0.0222,0.048125));
#7477=CARTESIAN_POINT('Origin',(-0.04655,-0.0222,0.053125));
#7478=CARTESIAN_POINT('Origin',(-0.04655,-0.0222,0.043125));
#7479=CARTESIAN_POINT('Origin',(-0.06655,-0.009975,0.02565));
#7480=CARTESIAN_POINT('Origin',(-0.06655,-0.009975,0.02565));
#7481=CARTESIAN_POINT('Origin',(-0.06655,-0.0122,0.061125));
#7482=CARTESIAN_POINT('Origin',(-0.06655,-0.00775,0.061125));
#7483=CARTESIAN_POINT('Origin',(-0.06655,-0.00775,-0.009825));
#7484=CARTESIAN_POINT('Origin',(-0.06655,-0.0122,-0.009825));
#7485=CARTESIAN_POINT('Origin',(-0.05755,-0.0272,0.02565));
#7486=CARTESIAN_POINT('',(-0.0622553825561797,-0.0272,0.008175));
#7487=CARTESIAN_POINT('',(-0.0685499999998011,-0.0271999999999999,0.00817500000000003));
#7488=CARTESIAN_POINT('',(-0.05755,-0.0272,0.0218));
#7489=CARTESIAN_POINT('Origin',(-0.05755,-0.0272,0.014175));
#7490=CARTESIAN_POINT('',(-0.0528446174438203,-0.0272,0.008175));
#7491=CARTESIAN_POINT('Origin',(-0.05755,-0.0272,0.014175));
#7492=CARTESIAN_POINT('',(-0.04655,-0.0272,0.008175));
#7493=CARTESIAN_POINT('',(-0.0528446174438203,-0.0272,0.043125));
#7494=CARTESIAN_POINT('',(-0.05755,-0.0272,0.043125));
#7495=CARTESIAN_POINT('',(-0.0622553825561797,-0.0272,0.043125));
#7496=CARTESIAN_POINT('Origin',(-0.05755,-0.0272,0.037125));
#7497=CARTESIAN_POINT('',(-0.0685499999998011,-0.0272,0.043125));
#7498=CARTESIAN_POINT('Origin',(-0.05755,-0.0022,0.037125));
#7499=CARTESIAN_POINT('',(-0.05755,-0.0269285700798444,0.04475));
#7500=CARTESIAN_POINT('',(-0.05755,-0.0022,0.04475));
#7501=CARTESIAN_POINT('Ctrl Pts',(-0.0622553825561797,-0.0272,0.043125));
#7502=CARTESIAN_POINT('Ctrl Pts',(-0.0617185912965407,-0.0272,0.0435459680382359));
#7503=CARTESIAN_POINT('Ctrl Pts',(-0.0611100942808263,-0.027146490983882,
0.0439040351600042));
#7504=CARTESIAN_POINT('Ctrl Pts',(-0.0595292759370733,-0.0270066019492738,
0.0445577665669935));
#7505=CARTESIAN_POINT('Ctrl Pts',(-0.058511387005684,-0.0269285700798444,
0.04475));
#7506=CARTESIAN_POINT('Ctrl Pts',(-0.05755,-0.0269285700798444,0.04475));
#7507=CARTESIAN_POINT('Ctrl Pts',(-0.05755,-0.0269285700798444,0.04475));
#7508=CARTESIAN_POINT('Ctrl Pts',(-0.056588612994316,-0.0269285700798444,
0.04475));
#7509=CARTESIAN_POINT('Ctrl Pts',(-0.0555707240629267,-0.0270066019492738,
0.0445577665669935));
#7510=CARTESIAN_POINT('Ctrl Pts',(-0.0539899057191737,-0.027146490983882,
0.0439040351600042));
#7511=CARTESIAN_POINT('Ctrl Pts',(-0.0533814087034593,-0.0272,0.0435459680382359));
#7512=CARTESIAN_POINT('Ctrl Pts',(-0.0528446174438203,-0.0272,0.043125));
#7513=CARTESIAN_POINT('Origin',(-0.05755,-0.0022,0.014175));
#7514=CARTESIAN_POINT('',(-0.05755,-0.0022,0.0218));
#7515=CARTESIAN_POINT('Ctrl Pts',(-0.0622553825561797,-0.0272,0.00817500000000001));
#7516=CARTESIAN_POINT('Ctrl Pts',(-0.0617185912965407,-0.0272,0.00775403196176415));
#7517=CARTESIAN_POINT('Ctrl Pts',(-0.0611100942808263,-0.027146490983882,
0.00739596483999584));
#7518=CARTESIAN_POINT('Ctrl Pts',(-0.0595292759370733,-0.0270066019492738,
0.00674223343300649));
#7519=CARTESIAN_POINT('Ctrl Pts',(-0.058511387005684,-0.0269285700798444,
0.00655));
#7520=CARTESIAN_POINT('Ctrl Pts',(-0.056588612994316,-0.0269285700798444,
0.00655));
#7521=CARTESIAN_POINT('Ctrl Pts',(-0.0555707240629267,-0.0270066019492738,
0.00674223343300649));
#7522=CARTESIAN_POINT('Ctrl Pts',(-0.0539899057191737,-0.027146490983882,
0.00739596483999584));
#7523=CARTESIAN_POINT('Ctrl Pts',(-0.0533814087034593,-0.0272,0.00775403196176415));
#7524=CARTESIAN_POINT('Ctrl Pts',(-0.0528446174438203,-0.0272,0.00817500000000001));
#7525=CARTESIAN_POINT('Origin',(-0.05755,-0.0222,0.008175));
#7526=CARTESIAN_POINT('',(-0.0685499999997944,-0.0221999999999999,0.00317500000000004));
#7527=CARTESIAN_POINT('Origin',(-0.05755,-0.0222,-0.001825));
#7528=CARTESIAN_POINT('Origin',(-0.05755,-0.0222,0.043125));
#7529=CARTESIAN_POINT('',(-0.0685499999997944,-0.0221999999999999,0.0481250000000001));
#7530=CARTESIAN_POINT('Origin',(-0.06655,-0.0222,0.053125));
#8922=UNCERTAINTY_MEASURE_WITH_UNIT(LENGTH_MEASURE(1.E-5),#8945,
'DISTANCE_ACCURACY_VALUE',
'Maximum model space distance between geometric entities at asserted c
onnectivities');
#8932=UNCERTAINTY_MEASURE_WITH_UNIT(LENGTH_MEASURE(1.E-5),#8945,
'DISTANCE_ACCURACY_VALUE',
'Maximum model space distance between geometric entities at asserted c
onnectivities');
#8934=(
GEOMETRIC_REPRESENTATION_CONTEXT(3)
GLOBAL_UNCERTAINTY_ASSIGNED_CONTEXT((#8922))
GLOBAL_UNIT_ASSIGNED_CONTEXT((#8945,#8946,#8947))
REPRESENTATION_CONTEXT('','3D')
);
#8944=(
GEOMETRIC_REPRESENTATION_CONTEXT(3)
GLOBAL_UNCERTAINTY_ASSIGNED_CONTEXT((#8932))
GLOBAL_UNIT_ASSIGNED_CONTEXT((#8945,#8946,#8947))
REPRESENTATION_CONTEXT('','3D')
);
#8945=(
LENGTH_UNIT()
NAMED_UNIT(*)
SI_UNIT($,.METRE.)
);
#8946=(
NAMED_UNIT(*)
PLANE_ANGLE_UNIT()
SI_UNIT($,.RADIAN.)
);
#8947=(
NAMED_UNIT(*)
SI_UNIT($,.STERADIAN.)
SOLID_ANGLE_UNIT()
);
#8949=SHAPE_DEFINITION_REPRESENTATION(#8960,#8993);
#8960=PRODUCT_DEFINITION_SHAPE('',$,#9005);
#8993=SHAPE_REPRESENTATION('',(#5260),#8934);
#9003=PRODUCT_DEFINITION_CONTEXT('part definition',#9038,'design');
#9005=PRODUCT_DEFINITION('End Cap Left','End Cap Left',#9016,#9003);
#9016=PRODUCT_DEFINITION_FORMATION('',$,#9041);
#9038=APPLICATION_CONTEXT('Managed model based 3d engineering');
#9039=PRODUCT_CONTEXT('part definition',#9038,'mechanical');
#9041=PRODUCT('End Cap Left','End Cap Left',
'LEGAL AND USAGE DISCLAIMER: this Data/Model is provided \X2\201C\X0\A
S IS\X2\201D\X0\ for informational and representational only. It is a 
geometric approximation and is NOT engineered, certified, or guarantee
d for dimensional accuracy, exact tolerances, or production-level prec
ision. Vendor disclaims all implied warranties including fitness for a
 particular purpose. DO NOT USE FOR DIRECT PHYSICAL MANUFACTURING, AUT
OMATED PRODUCTION, OR SAFETY-CRITICAL SYSTEMS without independent engi
neering verification and resolution of any design discrepancies.',(#9039));
#9052=PRESENTATION_STYLE_ASSIGNMENT((#9057));
#9057=SURFACE_STYLE_USAGE(.BOTH.,#9062);
#9062=SURFACE_SIDE_STYLE('',(#9067));
#9067=SURFACE_STYLE_FILL_AREA(#9072);
#9072=FILL_AREA_STYLE('Opaque(25,25,25)',(#9077));
#9077=FILL_AREA_STYLE_COLOUR('Opaque(25,25,25)',#9082);
#9082=COLOUR_RGB('Opaque(25,25,25)',0.0980392156862745,0.0980392156862745,
0.0980392156862745);
ENDSEC;
END-ISO-10303-21;
